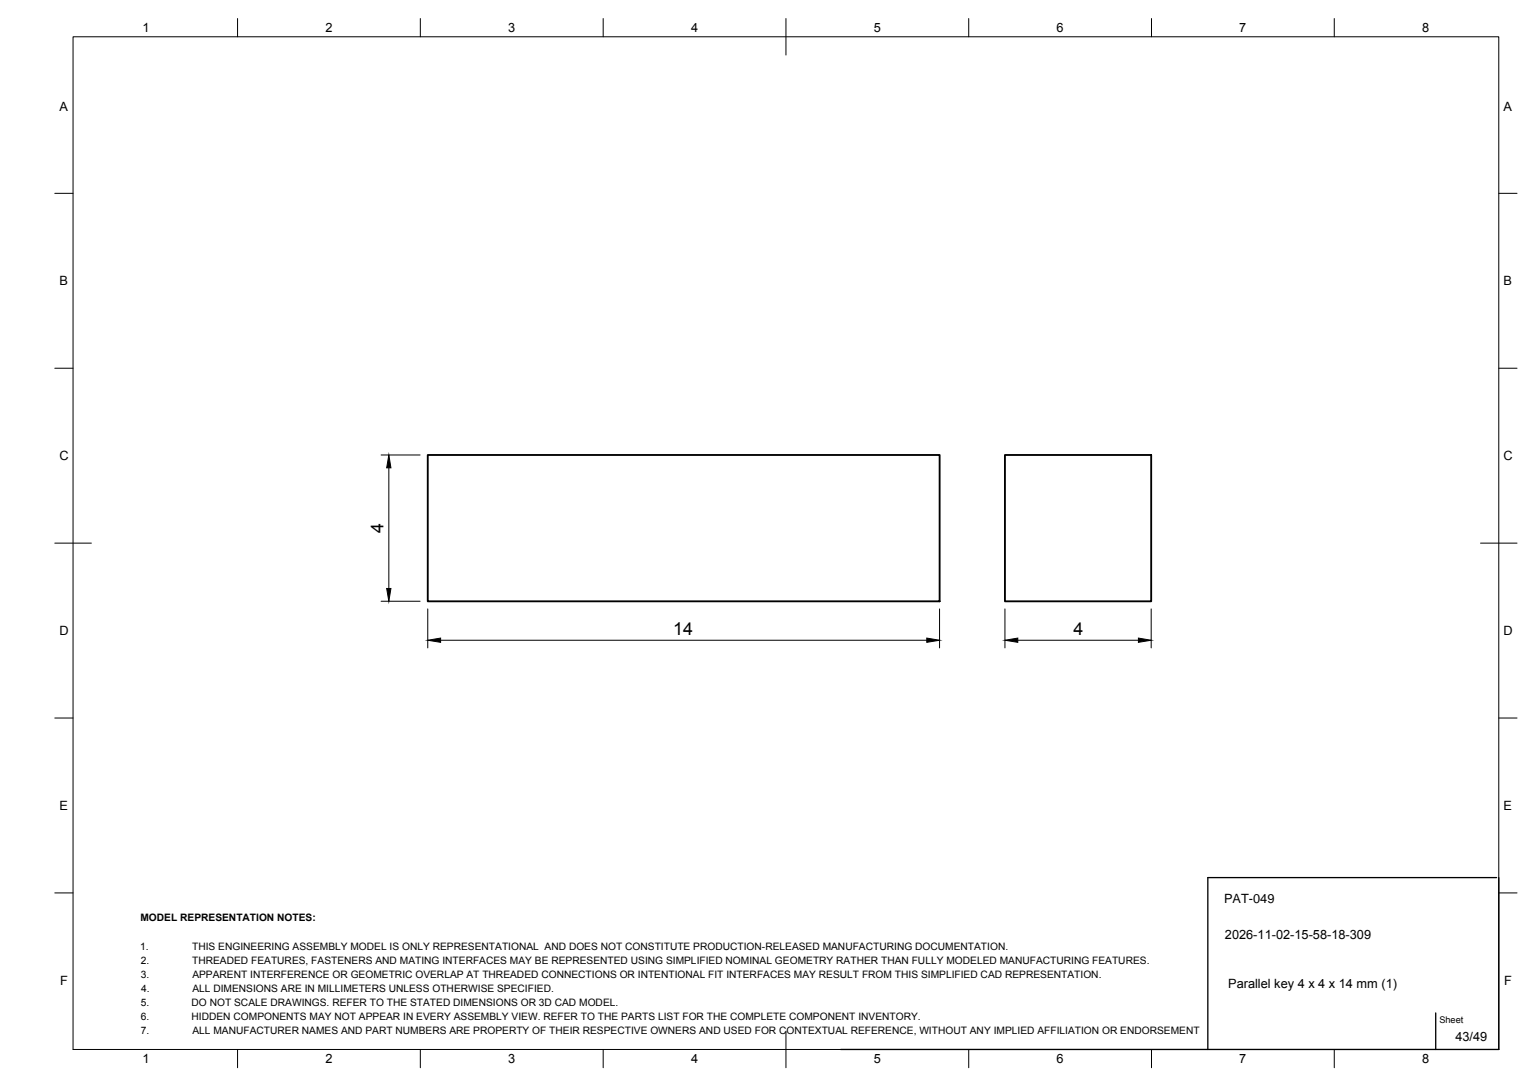
ISO-10303-21;
HEADER;
/* Generated by software containing ST-Developer
 * from STEP Tools, Inc. (www.steptools.com) 
 */

FILE_DESCRIPTION(
/* description */ ('Hand drill press frame (manual)'),
/* implementation_level */ '2;1');

FILE_NAME(
/* name */ 'Parallel key 4 x 4 x 14 mm (1).step',
/* time_stamp */ '2026-10-28T03:25:28-07:00',
/* author */ (''),
/* organization */ (''),
/* preprocessor_version */ 'ST-DEVELOPER v20.2',
/* originating_system */ 'Autodesk Translation Framework v15.17.0.0',
/* authorisation */ '');

FILE_SCHEMA (('AUTOMOTIVE_DESIGN { 1 0 10303 214 3 1 1 }'));
ENDSEC;

DATA;
#10=MECHANICAL_DESIGN_GEOMETRIC_PRESENTATION_REPRESENTATION('',(#661),#33299);
#564=SHAPE_REPRESENTATION_RELATIONSHIP('SRR','None',#33526,#609);
#609=ADVANCED_BREP_SHAPE_REPRESENTATION('',(#712),#33288);
#661=STYLED_ITEM('',(#33814),#712);
#712=MANIFOLD_SOLID_BREP('Body1',#12680);
#1266=PLANE('',#14077);
#1267=PLANE('',#14078);
#1268=PLANE('',#14079);
#1269=PLANE('',#14080);
#1270=PLANE('',#14081);
#1271=PLANE('',#14082);
#1867=FACE_OUTER_BOUND('',#2703,.T.);
#1868=FACE_OUTER_BOUND('',#2704,.T.);
#1869=FACE_OUTER_BOUND('',#2705,.T.);
#1870=FACE_OUTER_BOUND('',#2706,.T.);
#1871=FACE_OUTER_BOUND('',#2707,.T.);
#1872=FACE_OUTER_BOUND('',#2708,.T.);
#2703=EDGE_LOOP('',(#11003,#11004,#11005,#11006));
#2704=EDGE_LOOP('',(#11007,#11008,#11009,#11010));
#2705=EDGE_LOOP('',(#11011,#11012,#11013,#11014));
#2706=EDGE_LOOP('',(#11015,#11016,#11017,#11018));
#2707=EDGE_LOOP('',(#11019,#11020,#11021,#11022));
#2708=EDGE_LOOP('',(#11023,#11024,#11025,#11026));
#3828=LINE('',#21230,#4993);
#3829=LINE('',#21232,#4994);
#3830=LINE('',#21234,#4995);
#3831=LINE('',#21235,#4996);
#3832=LINE('',#21238,#4997);
#3833=LINE('',#21240,#4998);
#3834=LINE('',#21241,#4999);
#3835=LINE('',#21244,#5000);
#3836=LINE('',#21246,#5001);
#3837=LINE('',#21247,#5002);
#3838=LINE('',#21249,#5003);
#3839=LINE('',#21250,#5004);
#4993=VECTOR('',#17091,1.);
#4994=VECTOR('',#17092,1.);
#4995=VECTOR('',#17093,1.);
#4996=VECTOR('',#17094,1.);
#4997=VECTOR('',#17097,1.);
#4998=VECTOR('',#17098,1.);
#4999=VECTOR('',#17099,1.);
#5000=VECTOR('',#17102,1.);
#5001=VECTOR('',#17103,1.);
#5002=VECTOR('',#17104,1.);
#5003=VECTOR('',#17107,1.);
#5004=VECTOR('',#17108,1.);
#6481=VERTEX_POINT('',#21228);
#6482=VERTEX_POINT('',#21229);
#6483=VERTEX_POINT('',#21231);
#6484=VERTEX_POINT('',#21233);
#6485=VERTEX_POINT('',#21237);
#6486=VERTEX_POINT('',#21239);
#6487=VERTEX_POINT('',#21243);
#6488=VERTEX_POINT('',#21245);
#8030=EDGE_CURVE('',#6481,#6482,#3828,.T.);
#8031=EDGE_CURVE('',#6482,#6483,#3829,.T.);
#8032=EDGE_CURVE('',#6484,#6483,#3830,.T.);
#8033=EDGE_CURVE('',#6481,#6484,#3831,.T.);
#8034=EDGE_CURVE('',#6485,#6481,#3832,.T.);
#8035=EDGE_CURVE('',#6486,#6484,#3833,.T.);
#8036=EDGE_CURVE('',#6485,#6486,#3834,.T.);
#8037=EDGE_CURVE('',#6487,#6485,#3835,.T.);
#8038=EDGE_CURVE('',#6488,#6486,#3836,.T.);
#8039=EDGE_CURVE('',#6487,#6488,#3837,.T.);
#8040=EDGE_CURVE('',#6482,#6487,#3838,.T.);
#8041=EDGE_CURVE('',#6483,#6488,#3839,.T.);
#11003=ORIENTED_EDGE('',*,*,#8030,.T.);
#11004=ORIENTED_EDGE('',*,*,#8031,.T.);
#11005=ORIENTED_EDGE('',*,*,#8032,.F.);
#11006=ORIENTED_EDGE('',*,*,#8033,.F.);
#11007=ORIENTED_EDGE('',*,*,#8034,.T.);
#11008=ORIENTED_EDGE('',*,*,#8033,.T.);
#11009=ORIENTED_EDGE('',*,*,#8035,.F.);
#11010=ORIENTED_EDGE('',*,*,#8036,.F.);
#11011=ORIENTED_EDGE('',*,*,#8037,.T.);
#11012=ORIENTED_EDGE('',*,*,#8036,.T.);
#11013=ORIENTED_EDGE('',*,*,#8038,.F.);
#11014=ORIENTED_EDGE('',*,*,#8039,.F.);
#11015=ORIENTED_EDGE('',*,*,#8040,.T.);
#11016=ORIENTED_EDGE('',*,*,#8039,.T.);
#11017=ORIENTED_EDGE('',*,*,#8041,.F.);
#11018=ORIENTED_EDGE('',*,*,#8031,.F.);
#11019=ORIENTED_EDGE('',*,*,#8041,.T.);
#11020=ORIENTED_EDGE('',*,*,#8038,.T.);
#11021=ORIENTED_EDGE('',*,*,#8035,.T.);
#11022=ORIENTED_EDGE('',*,*,#8032,.T.);
#11023=ORIENTED_EDGE('',*,*,#8040,.F.);
#11024=ORIENTED_EDGE('',*,*,#8030,.F.);
#11025=ORIENTED_EDGE('',*,*,#8034,.F.);
#11026=ORIENTED_EDGE('',*,*,#8037,.F.);
#12476=ADVANCED_FACE('',(#1867),#1266,.T.);
#12477=ADVANCED_FACE('',(#1868),#1267,.T.);
#12478=ADVANCED_FACE('',(#1869),#1268,.T.);
#12479=ADVANCED_FACE('',(#1870),#1269,.T.);
#12480=ADVANCED_FACE('',(#1871),#1270,.T.);
#12481=ADVANCED_FACE('',(#1872),#1271,.F.);
#12680=CLOSED_SHELL('',(#12476,#12477,#12478,#12479,#12480,#12481));
#14076=AXIS2_PLACEMENT_3D('',#21226,#17087,#17088);
#14077=AXIS2_PLACEMENT_3D('',#21227,#17089,#17090);
#14078=AXIS2_PLACEMENT_3D('',#21236,#17095,#17096);
#14079=AXIS2_PLACEMENT_3D('',#21242,#17100,#17101);
#14080=AXIS2_PLACEMENT_3D('',#21248,#17105,#17106);
#14081=AXIS2_PLACEMENT_3D('',#21251,#17109,#17110);
#14082=AXIS2_PLACEMENT_3D('',#21252,#17111,#17112);
#17087=DIRECTION('axis',(0.,0.,1.));
#17088=DIRECTION('refdir',(1.,0.,0.));
#17089=DIRECTION('center_axis',(0.,1.,0.));
#17090=DIRECTION('ref_axis',(-1.,0.,0.));
#17091=DIRECTION('',(-1.,0.,0.));
#17092=DIRECTION('',(0.,0.,1.));
#17093=DIRECTION('',(-1.,0.,0.));
#17094=DIRECTION('',(0.,0.,1.));
#17095=DIRECTION('center_axis',(1.,0.,0.));
#17096=DIRECTION('ref_axis',(0.,1.,0.));
#17097=DIRECTION('',(0.,1.,0.));
#17098=DIRECTION('',(0.,1.,0.));
#17099=DIRECTION('',(0.,0.,1.));
#17100=DIRECTION('center_axis',(0.,-1.,0.));
#17101=DIRECTION('ref_axis',(1.,0.,0.));
#17102=DIRECTION('',(1.,0.,0.));
#17103=DIRECTION('',(1.,0.,0.));
#17104=DIRECTION('',(0.,0.,1.));
#17105=DIRECTION('center_axis',(-1.,0.,0.));
#17106=DIRECTION('ref_axis',(0.,-1.,0.));
#17107=DIRECTION('',(0.,-1.,0.));
#17108=DIRECTION('',(0.,-1.,0.));
#17109=DIRECTION('center_axis',(0.,0.,1.));
#17110=DIRECTION('ref_axis',(1.,0.,0.));
#17111=DIRECTION('center_axis',(0.,0.,1.));
#17112=DIRECTION('ref_axis',(1.,0.,0.));
#21226=CARTESIAN_POINT('',(0.,0.,0.));
#21227=CARTESIAN_POINT('Origin',(-2.5,6.9,19.8));
#21228=CARTESIAN_POINT('',(-2.5,6.9,19.8));
#21229=CARTESIAN_POINT('',(-2.9,6.9,19.8));
#21230=CARTESIAN_POINT('',(-2.5,6.9,19.8));
#21231=CARTESIAN_POINT('',(-2.9,6.9,20.2));
#21232=CARTESIAN_POINT('',(-2.9,6.9,19.8));
#21233=CARTESIAN_POINT('',(-2.5,6.9,20.2));
#21234=CARTESIAN_POINT('',(-2.5,6.9,20.2));
#21235=CARTESIAN_POINT('',(-2.5,6.9,19.8));
#21236=CARTESIAN_POINT('Origin',(-2.5,5.5,19.8));
#21237=CARTESIAN_POINT('',(-2.5,5.5,19.8));
#21238=CARTESIAN_POINT('',(-2.5,5.5,19.8));
#21239=CARTESIAN_POINT('',(-2.5,5.5,20.2));
#21240=CARTESIAN_POINT('',(-2.5,5.5,20.2));
#21241=CARTESIAN_POINT('',(-2.5,5.5,19.8));
#21242=CARTESIAN_POINT('Origin',(-2.9,5.5,19.8));
#21243=CARTESIAN_POINT('',(-2.9,5.5,19.8));
#21244=CARTESIAN_POINT('',(-2.9,5.5,19.8));
#21245=CARTESIAN_POINT('',(-2.9,5.5,20.2));
#21246=CARTESIAN_POINT('',(-2.9,5.5,20.2));
#21247=CARTESIAN_POINT('',(-2.9,5.5,19.8));
#21248=CARTESIAN_POINT('Origin',(-2.9,6.9,19.8));
#21249=CARTESIAN_POINT('',(-2.9,6.9,19.8));
#21250=CARTESIAN_POINT('',(-2.9,6.9,20.2));
#21251=CARTESIAN_POINT('Origin',(-2.7,6.2,20.2));
#21252=CARTESIAN_POINT('Origin',(-2.7,6.2,19.8));
#33236=UNCERTAINTY_MEASURE_WITH_UNIT(LENGTH_MEASURE(0.001),#33300,
'DISTANCE_ACCURACY_VALUE',
'Maximum model space distance between geometric entities at asserted c
onnectivities');
#33247=UNCERTAINTY_MEASURE_WITH_UNIT(LENGTH_MEASURE(0.001),#33300,
'DISTANCE_ACCURACY_VALUE',
'Maximum model space distance between geometric entities at asserted c
onnectivities');
#33288=(
GEOMETRIC_REPRESENTATION_CONTEXT(3)
GLOBAL_UNCERTAINTY_ASSIGNED_CONTEXT((#33236))
GLOBAL_UNIT_ASSIGNED_CONTEXT((#33300,#33302,#33303))
REPRESENTATION_CONTEXT('','3D')
);
#33299=(
GEOMETRIC_REPRESENTATION_CONTEXT(3)
GLOBAL_UNCERTAINTY_ASSIGNED_CONTEXT((#33247))
GLOBAL_UNIT_ASSIGNED_CONTEXT((#33300,#33302,#33303))
REPRESENTATION_CONTEXT('','3D')
);
#33300=(
LENGTH_UNIT()
NAMED_UNIT(*)
SI_UNIT(.CENTI.,.METRE.)
);
#33302=(
NAMED_UNIT(*)
PLANE_ANGLE_UNIT()
SI_UNIT($,.RADIAN.)
);
#33303=(
NAMED_UNIT(*)
SI_UNIT($,.STERADIAN.)
SOLID_ANGLE_UNIT()
);
#33344=SHAPE_DEFINITION_REPRESENTATION(#33406,#33526);
#33406=PRODUCT_DEFINITION_SHAPE('',$,#33578);
#33526=SHAPE_REPRESENTATION('',(#14076),#33288);
#33537=PRODUCT_DEFINITION_CONTEXT('part definition',#33692,'design');
#33578=PRODUCT_DEFINITION('Parallel key 4 x 4 x 14 mm (1)',
'Parallel key 4 x 4 x 14 mm (1)',#33629,#33537);
#33629=PRODUCT_DEFINITION_FORMATION('',$,#33734);
#33692=APPLICATION_CONTEXT(
'Core Data for Automotive Mechanical Design Process');
#33693=PRODUCT_CONTEXT('part definition',#33692,'mechanical');
#33734=PRODUCT('Parallel key 4 x 4 x 14 mm (1)',
'Parallel key 4 x 4 x 14 mm (1)','Parallel key 4 x 4 x 14 mm (1)',(#33693));
#33808=COLOUR_RGB('Grey',0.48,0.52,0.57);
#33809=FILL_AREA_STYLE_COLOUR('',#33808);
#33810=FILL_AREA_STYLE('',(#33809));
#33811=SURFACE_STYLE_FILL_AREA(#33810);
#33812=SURFACE_SIDE_STYLE('',(#33811));
#33813=SURFACE_STYLE_USAGE(.BOTH.,#33812);
#33814=PRESENTATION_STYLE_ASSIGNMENT((#33813));
ENDSEC;
END-ISO-10303-21;
